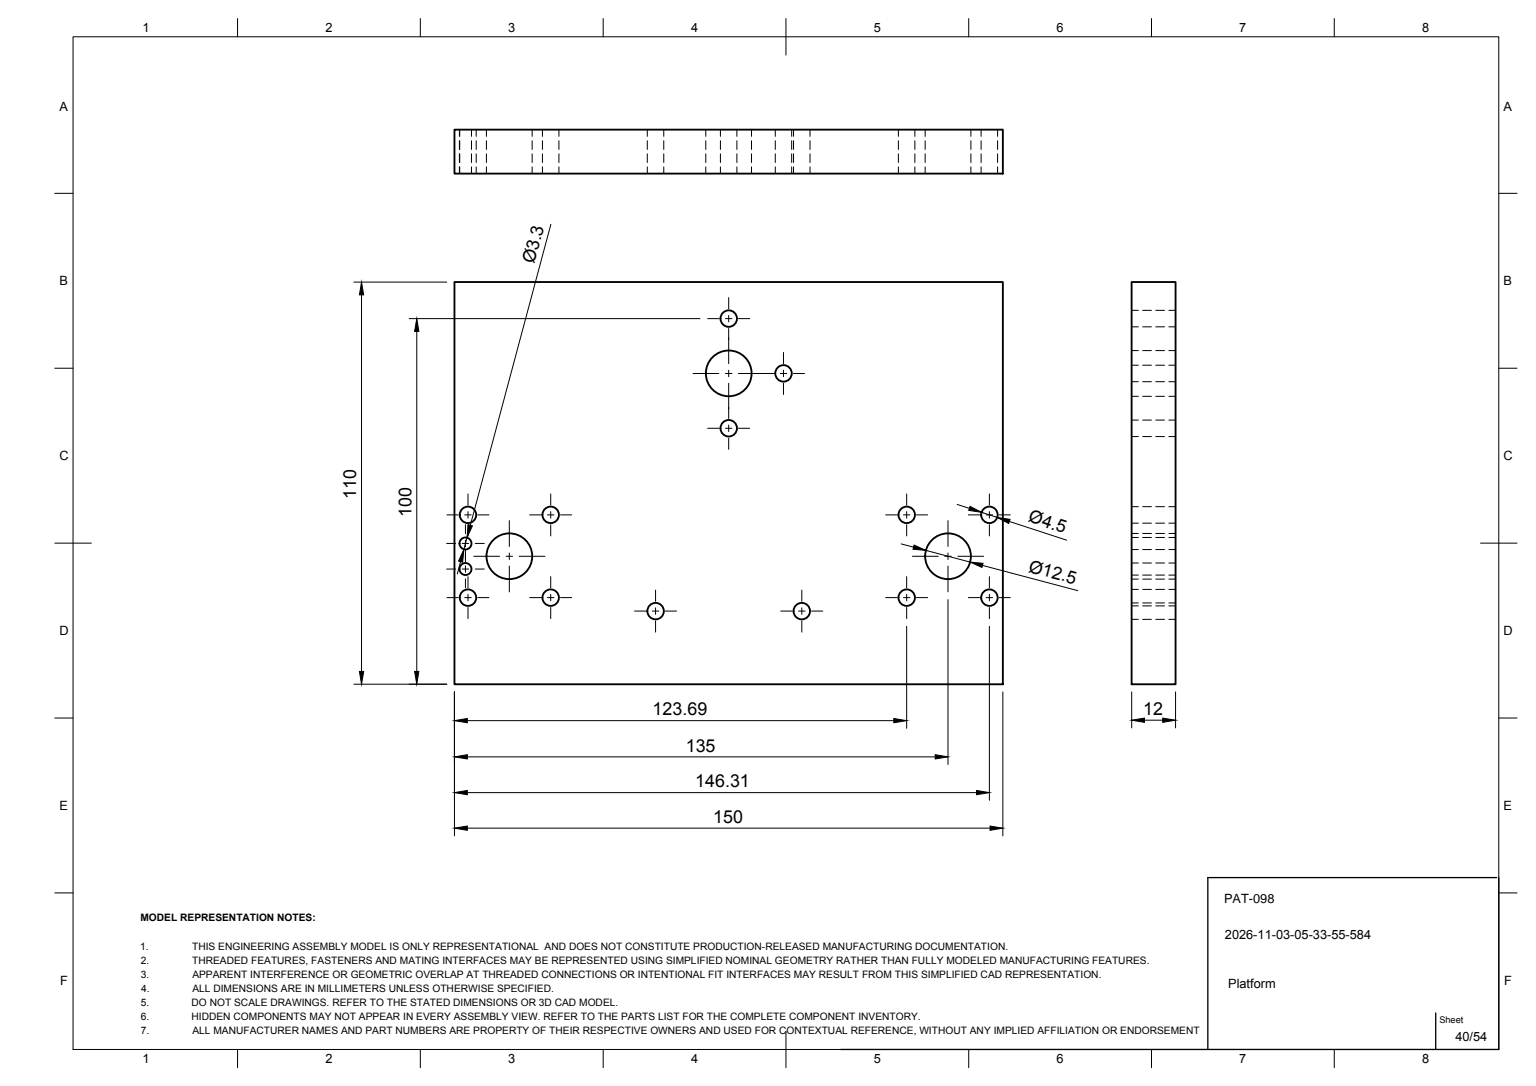
ISO-10303-21;
HEADER;
/* Generated by software containing ST-Developer
 * from STEP Tools, Inc. (www.steptools.com) 
 */

FILE_DESCRIPTION(
/* description */ ('Spring compression tester'),
/* implementation_level */ '2;1');

FILE_NAME(
/* name */ 'Platform.step',
/* time_stamp */ '2026-10-28T03:24:11-07:00',
/* author */ (''),
/* organization */ (''),
/* preprocessor_version */ 'ST-DEVELOPER v20.2',
/* originating_system */ 'Autodesk Translation Framework v15.17.0.0',
/* authorisation */ '');

FILE_SCHEMA (('AUTOMOTIVE_DESIGN { 1 0 10303 214 3 1 1 }'));
ENDSEC;

DATA;
#10=MECHANICAL_DESIGN_GEOMETRIC_PRESENTATION_REPRESENTATION('',(#1158),#43521);
#1023=SHAPE_REPRESENTATION_RELATIONSHIP('SRR','None',#43838,#1083);
#1083=ADVANCED_BREP_SHAPE_REPRESENTATION('',(#1229),#43498);
#1158=STYLED_ITEM('',(#44188),#1229);
#1229=MANIFOLD_SOLID_BREP('Body1',#18599);
#1477=FACE_BOUND('',#4122,.T.);
#1478=FACE_BOUND('',#4123,.T.);
#1479=FACE_BOUND('',#4124,.T.);
#1480=FACE_BOUND('',#4125,.T.);
#1481=FACE_BOUND('',#4126,.T.);
#1482=FACE_BOUND('',#4127,.T.);
#1483=FACE_BOUND('',#4128,.T.);
#1484=FACE_BOUND('',#4129,.T.);
#1485=FACE_BOUND('',#4130,.T.);
#1486=FACE_BOUND('',#4131,.T.);
#1487=FACE_BOUND('',#4132,.T.);
#1488=FACE_BOUND('',#4133,.T.);
#1489=FACE_BOUND('',#4134,.T.);
#1490=FACE_BOUND('',#4135,.T.);
#1491=FACE_BOUND('',#4136,.T.);
#1492=FACE_BOUND('',#4137,.T.);
#1493=FACE_BOUND('',#4138,.T.);
#1494=FACE_BOUND('',#4139,.T.);
#1495=FACE_BOUND('',#4141,.T.);
#1496=FACE_BOUND('',#4142,.T.);
#1497=FACE_BOUND('',#4143,.T.);
#1498=FACE_BOUND('',#4144,.T.);
#1499=FACE_BOUND('',#4145,.T.);
#1500=FACE_BOUND('',#4146,.T.);
#1501=FACE_BOUND('',#4147,.T.);
#1502=FACE_BOUND('',#4148,.T.);
#1503=FACE_BOUND('',#4149,.T.);
#1504=FACE_BOUND('',#4150,.T.);
#1505=FACE_BOUND('',#4151,.T.);
#1506=FACE_BOUND('',#4152,.T.);
#1507=FACE_BOUND('',#4153,.T.);
#1508=FACE_BOUND('',#4154,.T.);
#1509=FACE_BOUND('',#4155,.T.);
#1510=FACE_BOUND('',#4156,.T.);
#1511=FACE_BOUND('',#4157,.T.);
#1512=FACE_BOUND('',#4158,.T.);
#2024=PLANE('',#20482);
#2025=PLANE('',#20483);
#2026=PLANE('',#20484);
#2027=PLANE('',#20485);
#2028=PLANE('',#20486);
#2029=PLANE('',#20487);
#2822=FACE_OUTER_BOUND('',#4099,.T.);
#2823=FACE_OUTER_BOUND('',#4100,.T.);
#2824=FACE_OUTER_BOUND('',#4101,.T.);
#2825=FACE_OUTER_BOUND('',#4102,.T.);
#2826=FACE_OUTER_BOUND('',#4103,.T.);
#2827=FACE_OUTER_BOUND('',#4104,.T.);
#2828=FACE_OUTER_BOUND('',#4105,.T.);
#2829=FACE_OUTER_BOUND('',#4106,.T.);
#2830=FACE_OUTER_BOUND('',#4107,.T.);
#2831=FACE_OUTER_BOUND('',#4108,.T.);
#2832=FACE_OUTER_BOUND('',#4109,.T.);
#2833=FACE_OUTER_BOUND('',#4110,.T.);
#2834=FACE_OUTER_BOUND('',#4111,.T.);
#2835=FACE_OUTER_BOUND('',#4112,.T.);
#2836=FACE_OUTER_BOUND('',#4113,.T.);
#2837=FACE_OUTER_BOUND('',#4114,.T.);
#2838=FACE_OUTER_BOUND('',#4115,.T.);
#2839=FACE_OUTER_BOUND('',#4116,.T.);
#2840=FACE_OUTER_BOUND('',#4117,.T.);
#2841=FACE_OUTER_BOUND('',#4118,.T.);
#2842=FACE_OUTER_BOUND('',#4119,.T.);
#2843=FACE_OUTER_BOUND('',#4120,.T.);
#2844=FACE_OUTER_BOUND('',#4121,.T.);
#2845=FACE_OUTER_BOUND('',#4140,.T.);
#4099=EDGE_LOOP('',(#15129,#15130,#15131,#15132));
#4100=EDGE_LOOP('',(#15133,#15134,#15135,#15136));
#4101=EDGE_LOOP('',(#15137,#15138,#15139,#15140));
#4102=EDGE_LOOP('',(#15141,#15142,#15143,#15144));
#4103=EDGE_LOOP('',(#15145,#15146,#15147,#15148));
#4104=EDGE_LOOP('',(#15149,#15150,#15151,#15152));
#4105=EDGE_LOOP('',(#15153,#15154,#15155,#15156));
#4106=EDGE_LOOP('',(#15157,#15158,#15159,#15160));
#4107=EDGE_LOOP('',(#15161,#15162,#15163,#15164));
#4108=EDGE_LOOP('',(#15165,#15166,#15167,#15168));
#4109=EDGE_LOOP('',(#15169,#15170,#15171,#15172));
#4110=EDGE_LOOP('',(#15173,#15174,#15175,#15176));
#4111=EDGE_LOOP('',(#15177,#15178,#15179,#15180));
#4112=EDGE_LOOP('',(#15181,#15182,#15183,#15184));
#4113=EDGE_LOOP('',(#15185,#15186,#15187,#15188));
#4114=EDGE_LOOP('',(#15189,#15190,#15191,#15192));
#4115=EDGE_LOOP('',(#15193,#15194,#15195,#15196));
#4116=EDGE_LOOP('',(#15197,#15198,#15199,#15200));
#4117=EDGE_LOOP('',(#15201,#15202,#15203,#15204));
#4118=EDGE_LOOP('',(#15205,#15206,#15207,#15208));
#4119=EDGE_LOOP('',(#15209,#15210,#15211,#15212));
#4120=EDGE_LOOP('',(#15213,#15214,#15215,#15216));
#4121=EDGE_LOOP('',(#15217,#15218,#15219,#15220));
#4122=EDGE_LOOP('',(#15221));
#4123=EDGE_LOOP('',(#15222));
#4124=EDGE_LOOP('',(#15223));
#4125=EDGE_LOOP('',(#15224));
#4126=EDGE_LOOP('',(#15225));
#4127=EDGE_LOOP('',(#15226));
#4128=EDGE_LOOP('',(#15227));
#4129=EDGE_LOOP('',(#15228));
#4130=EDGE_LOOP('',(#15229));
#4131=EDGE_LOOP('',(#15230));
#4132=EDGE_LOOP('',(#15231));
#4133=EDGE_LOOP('',(#15232));
#4134=EDGE_LOOP('',(#15233));
#4135=EDGE_LOOP('',(#15234));
#4136=EDGE_LOOP('',(#15235));
#4137=EDGE_LOOP('',(#15236));
#4138=EDGE_LOOP('',(#15237));
#4139=EDGE_LOOP('',(#15238));
#4140=EDGE_LOOP('',(#15239,#15240,#15241,#15242));
#4141=EDGE_LOOP('',(#15243));
#4142=EDGE_LOOP('',(#15244));
#4143=EDGE_LOOP('',(#15245));
#4144=EDGE_LOOP('',(#15246));
#4145=EDGE_LOOP('',(#15247));
#4146=EDGE_LOOP('',(#15248));
#4147=EDGE_LOOP('',(#15249));
#4148=EDGE_LOOP('',(#15250));
#4149=EDGE_LOOP('',(#15251));
#4150=EDGE_LOOP('',(#15252));
#4151=EDGE_LOOP('',(#15253));
#4152=EDGE_LOOP('',(#15254));
#4153=EDGE_LOOP('',(#15255));
#4154=EDGE_LOOP('',(#15256));
#4155=EDGE_LOOP('',(#15257));
#4156=EDGE_LOOP('',(#15258));
#4157=EDGE_LOOP('',(#15259));
#4158=EDGE_LOOP('',(#15260));
#5593=LINE('',#30233,#7025);
#5594=LINE('',#30239,#7026);
#5595=LINE('',#30245,#7027);
#5596=LINE('',#30251,#7028);
#5597=LINE('',#30257,#7029);
#5598=LINE('',#30263,#7030);
#5599=LINE('',#30269,#7031);
#5600=LINE('',#30275,#7032);
#5601=LINE('',#30281,#7033);
#5602=LINE('',#30287,#7034);
#5603=LINE('',#30293,#7035);
#5604=LINE('',#30299,#7036);
#5605=LINE('',#30305,#7037);
#5606=LINE('',#30311,#7038);
#5607=LINE('',#30317,#7039);
#5608=LINE('',#30323,#7040);
#5609=LINE('',#30329,#7041);
#5610=LINE('',#30335,#7042);
#5611=LINE('',#30340,#7043);
#5612=LINE('',#30342,#7044);
#5613=LINE('',#30344,#7045);
#5614=LINE('',#30345,#7046);
#5615=LINE('',#30348,#7047);
#5616=LINE('',#30350,#7048);
#5617=LINE('',#30351,#7049);
#5618=LINE('',#30354,#7050);
#5619=LINE('',#30356,#7051);
#5620=LINE('',#30357,#7052);
#5621=LINE('',#30359,#7053);
#5622=LINE('',#30360,#7054);
#7025=VECTOR('',#24475,0.165);
#7026=VECTOR('',#24482,0.165);
#7027=VECTOR('',#24489,0.225);
#7028=VECTOR('',#24496,0.225);
#7029=VECTOR('',#24503,0.225);
#7030=VECTOR('',#24510,0.225);
#7031=VECTOR('',#24517,0.225);
#7032=VECTOR('',#24524,0.225);
#7033=VECTOR('',#24531,0.225);
#7034=VECTOR('',#24538,0.225);
#7035=VECTOR('',#24545,0.225);
#7036=VECTOR('',#24552,0.225);
#7037=VECTOR('',#24559,0.225);
#7038=VECTOR('',#24566,0.225);
#7039=VECTOR('',#24573,0.225);
#7040=VECTOR('',#24580,0.625);
#7041=VECTOR('',#24587,0.625);
#7042=VECTOR('',#24594,0.625);
#7043=VECTOR('',#24599,1.);
#7044=VECTOR('',#24600,1.);
#7045=VECTOR('',#24601,1.);
#7046=VECTOR('',#24602,1.);
#7047=VECTOR('',#24605,1.);
#7048=VECTOR('',#24606,1.);
#7049=VECTOR('',#24607,1.);
#7050=VECTOR('',#24610,1.);
#7051=VECTOR('',#24611,1.);
#7052=VECTOR('',#24612,1.);
#7053=VECTOR('',#24615,1.);
#7054=VECTOR('',#24616,1.);
#7905=CIRCLE('',#20429,0.165);
#7906=CIRCLE('',#20430,0.165);
#7907=CIRCLE('',#20432,0.165);
#7908=CIRCLE('',#20433,0.165);
#7909=CIRCLE('',#20435,0.225);
#7910=CIRCLE('',#20436,0.225);
#7911=CIRCLE('',#20438,0.225);
#7912=CIRCLE('',#20439,0.225);
#7913=CIRCLE('',#20441,0.225);
#7914=CIRCLE('',#20442,0.225);
#7915=CIRCLE('',#20444,0.225);
#7916=CIRCLE('',#20445,0.225);
#7917=CIRCLE('',#20447,0.225);
#7918=CIRCLE('',#20448,0.225);
#7919=CIRCLE('',#20450,0.225);
#7920=CIRCLE('',#20451,0.225);
#7921=CIRCLE('',#20453,0.225);
#7922=CIRCLE('',#20454,0.225);
#7923=CIRCLE('',#20456,0.225);
#7924=CIRCLE('',#20457,0.225);
#7925=CIRCLE('',#20459,0.225);
#7926=CIRCLE('',#20460,0.225);
#7927=CIRCLE('',#20462,0.225);
#7928=CIRCLE('',#20463,0.225);
#7929=CIRCLE('',#20465,0.225);
#7930=CIRCLE('',#20466,0.225);
#7931=CIRCLE('',#20468,0.225);
#7932=CIRCLE('',#20469,0.225);
#7933=CIRCLE('',#20471,0.225);
#7934=CIRCLE('',#20472,0.225);
#7935=CIRCLE('',#20474,0.625);
#7936=CIRCLE('',#20475,0.625);
#7937=CIRCLE('',#20477,0.625);
#7938=CIRCLE('',#20478,0.625);
#7939=CIRCLE('',#20480,0.625);
#7940=CIRCLE('',#20481,0.625);
#9118=VERTEX_POINT('',#30230);
#9119=VERTEX_POINT('',#30232);
#9120=VERTEX_POINT('',#30236);
#9121=VERTEX_POINT('',#30238);
#9122=VERTEX_POINT('',#30242);
#9123=VERTEX_POINT('',#30244);
#9124=VERTEX_POINT('',#30248);
#9125=VERTEX_POINT('',#30250);
#9126=VERTEX_POINT('',#30254);
#9127=VERTEX_POINT('',#30256);
#9128=VERTEX_POINT('',#30260);
#9129=VERTEX_POINT('',#30262);
#9130=VERTEX_POINT('',#30266);
#9131=VERTEX_POINT('',#30268);
#9132=VERTEX_POINT('',#30272);
#9133=VERTEX_POINT('',#30274);
#9134=VERTEX_POINT('',#30278);
#9135=VERTEX_POINT('',#30280);
#9136=VERTEX_POINT('',#30284);
#9137=VERTEX_POINT('',#30286);
#9138=VERTEX_POINT('',#30290);
#9139=VERTEX_POINT('',#30292);
#9140=VERTEX_POINT('',#30296);
#9141=VERTEX_POINT('',#30298);
#9142=VERTEX_POINT('',#30302);
#9143=VERTEX_POINT('',#30304);
#9144=VERTEX_POINT('',#30308);
#9145=VERTEX_POINT('',#30310);
#9146=VERTEX_POINT('',#30314);
#9147=VERTEX_POINT('',#30316);
#9148=VERTEX_POINT('',#30320);
#9149=VERTEX_POINT('',#30322);
#9150=VERTEX_POINT('',#30326);
#9151=VERTEX_POINT('',#30328);
#9152=VERTEX_POINT('',#30332);
#9153=VERTEX_POINT('',#30334);
#9154=VERTEX_POINT('',#30338);
#9155=VERTEX_POINT('',#30339);
#9156=VERTEX_POINT('',#30341);
#9157=VERTEX_POINT('',#30343);
#9158=VERTEX_POINT('',#30347);
#9159=VERTEX_POINT('',#30349);
#9160=VERTEX_POINT('',#30353);
#9161=VERTEX_POINT('',#30355);
#11229=EDGE_CURVE('',#9118,#9118,#7905,.T.);
#11230=EDGE_CURVE('',#9118,#9119,#5593,.T.);
#11231=EDGE_CURVE('',#9119,#9119,#7906,.T.);
#11232=EDGE_CURVE('',#9120,#9120,#7907,.T.);
#11233=EDGE_CURVE('',#9120,#9121,#5594,.T.);
#11234=EDGE_CURVE('',#9121,#9121,#7908,.T.);
#11235=EDGE_CURVE('',#9122,#9122,#7909,.T.);
#11236=EDGE_CURVE('',#9122,#9123,#5595,.T.);
#11237=EDGE_CURVE('',#9123,#9123,#7910,.T.);
#11238=EDGE_CURVE('',#9124,#9124,#7911,.T.);
#11239=EDGE_CURVE('',#9124,#9125,#5596,.T.);
#11240=EDGE_CURVE('',#9125,#9125,#7912,.T.);
#11241=EDGE_CURVE('',#9126,#9126,#7913,.T.);
#11242=EDGE_CURVE('',#9126,#9127,#5597,.T.);
#11243=EDGE_CURVE('',#9127,#9127,#7914,.T.);
#11244=EDGE_CURVE('',#9128,#9128,#7915,.T.);
#11245=EDGE_CURVE('',#9128,#9129,#5598,.T.);
#11246=EDGE_CURVE('',#9129,#9129,#7916,.T.);
#11247=EDGE_CURVE('',#9130,#9130,#7917,.T.);
#11248=EDGE_CURVE('',#9130,#9131,#5599,.T.);
#11249=EDGE_CURVE('',#9131,#9131,#7918,.T.);
#11250=EDGE_CURVE('',#9132,#9132,#7919,.T.);
#11251=EDGE_CURVE('',#9132,#9133,#5600,.T.);
#11252=EDGE_CURVE('',#9133,#9133,#7920,.T.);
#11253=EDGE_CURVE('',#9134,#9134,#7921,.T.);
#11254=EDGE_CURVE('',#9134,#9135,#5601,.T.);
#11255=EDGE_CURVE('',#9135,#9135,#7922,.T.);
#11256=EDGE_CURVE('',#9136,#9136,#7923,.T.);
#11257=EDGE_CURVE('',#9136,#9137,#5602,.T.);
#11258=EDGE_CURVE('',#9137,#9137,#7924,.T.);
#11259=EDGE_CURVE('',#9138,#9138,#7925,.T.);
#11260=EDGE_CURVE('',#9138,#9139,#5603,.T.);
#11261=EDGE_CURVE('',#9139,#9139,#7926,.T.);
#11262=EDGE_CURVE('',#9140,#9140,#7927,.T.);
#11263=EDGE_CURVE('',#9140,#9141,#5604,.T.);
#11264=EDGE_CURVE('',#9141,#9141,#7928,.T.);
#11265=EDGE_CURVE('',#9142,#9142,#7929,.T.);
#11266=EDGE_CURVE('',#9142,#9143,#5605,.T.);
#11267=EDGE_CURVE('',#9143,#9143,#7930,.T.);
#11268=EDGE_CURVE('',#9144,#9144,#7931,.T.);
#11269=EDGE_CURVE('',#9144,#9145,#5606,.T.);
#11270=EDGE_CURVE('',#9145,#9145,#7932,.T.);
#11271=EDGE_CURVE('',#9146,#9146,#7933,.T.);
#11272=EDGE_CURVE('',#9146,#9147,#5607,.T.);
#11273=EDGE_CURVE('',#9147,#9147,#7934,.T.);
#11274=EDGE_CURVE('',#9148,#9148,#7935,.T.);
#11275=EDGE_CURVE('',#9148,#9149,#5608,.T.);
#11276=EDGE_CURVE('',#9149,#9149,#7936,.T.);
#11277=EDGE_CURVE('',#9150,#9150,#7937,.T.);
#11278=EDGE_CURVE('',#9150,#9151,#5609,.T.);
#11279=EDGE_CURVE('',#9151,#9151,#7938,.T.);
#11280=EDGE_CURVE('',#9152,#9152,#7939,.T.);
#11281=EDGE_CURVE('',#9152,#9153,#5610,.T.);
#11282=EDGE_CURVE('',#9153,#9153,#7940,.T.);
#11283=EDGE_CURVE('',#9154,#9155,#5611,.T.);
#11284=EDGE_CURVE('',#9155,#9156,#5612,.T.);
#11285=EDGE_CURVE('',#9157,#9156,#5613,.T.);
#11286=EDGE_CURVE('',#9154,#9157,#5614,.T.);
#11287=EDGE_CURVE('',#9158,#9154,#5615,.T.);
#11288=EDGE_CURVE('',#9159,#9157,#5616,.T.);
#11289=EDGE_CURVE('',#9158,#9159,#5617,.T.);
#11290=EDGE_CURVE('',#9160,#9158,#5618,.T.);
#11291=EDGE_CURVE('',#9161,#9159,#5619,.T.);
#11292=EDGE_CURVE('',#9160,#9161,#5620,.T.);
#11293=EDGE_CURVE('',#9155,#9160,#5621,.T.);
#11294=EDGE_CURVE('',#9156,#9161,#5622,.T.);
#15129=ORIENTED_EDGE('',*,*,#11229,.F.);
#15130=ORIENTED_EDGE('',*,*,#11230,.T.);
#15131=ORIENTED_EDGE('',*,*,#11231,.F.);
#15132=ORIENTED_EDGE('',*,*,#11230,.F.);
#15133=ORIENTED_EDGE('',*,*,#11232,.F.);
#15134=ORIENTED_EDGE('',*,*,#11233,.T.);
#15135=ORIENTED_EDGE('',*,*,#11234,.F.);
#15136=ORIENTED_EDGE('',*,*,#11233,.F.);
#15137=ORIENTED_EDGE('',*,*,#11235,.F.);
#15138=ORIENTED_EDGE('',*,*,#11236,.T.);
#15139=ORIENTED_EDGE('',*,*,#11237,.F.);
#15140=ORIENTED_EDGE('',*,*,#11236,.F.);
#15141=ORIENTED_EDGE('',*,*,#11238,.F.);
#15142=ORIENTED_EDGE('',*,*,#11239,.T.);
#15143=ORIENTED_EDGE('',*,*,#11240,.F.);
#15144=ORIENTED_EDGE('',*,*,#11239,.F.);
#15145=ORIENTED_EDGE('',*,*,#11241,.F.);
#15146=ORIENTED_EDGE('',*,*,#11242,.T.);
#15147=ORIENTED_EDGE('',*,*,#11243,.F.);
#15148=ORIENTED_EDGE('',*,*,#11242,.F.);
#15149=ORIENTED_EDGE('',*,*,#11244,.F.);
#15150=ORIENTED_EDGE('',*,*,#11245,.T.);
#15151=ORIENTED_EDGE('',*,*,#11246,.F.);
#15152=ORIENTED_EDGE('',*,*,#11245,.F.);
#15153=ORIENTED_EDGE('',*,*,#11247,.F.);
#15154=ORIENTED_EDGE('',*,*,#11248,.T.);
#15155=ORIENTED_EDGE('',*,*,#11249,.F.);
#15156=ORIENTED_EDGE('',*,*,#11248,.F.);
#15157=ORIENTED_EDGE('',*,*,#11250,.F.);
#15158=ORIENTED_EDGE('',*,*,#11251,.T.);
#15159=ORIENTED_EDGE('',*,*,#11252,.F.);
#15160=ORIENTED_EDGE('',*,*,#11251,.F.);
#15161=ORIENTED_EDGE('',*,*,#11253,.F.);
#15162=ORIENTED_EDGE('',*,*,#11254,.T.);
#15163=ORIENTED_EDGE('',*,*,#11255,.F.);
#15164=ORIENTED_EDGE('',*,*,#11254,.F.);
#15165=ORIENTED_EDGE('',*,*,#11256,.F.);
#15166=ORIENTED_EDGE('',*,*,#11257,.T.);
#15167=ORIENTED_EDGE('',*,*,#11258,.F.);
#15168=ORIENTED_EDGE('',*,*,#11257,.F.);
#15169=ORIENTED_EDGE('',*,*,#11259,.F.);
#15170=ORIENTED_EDGE('',*,*,#11260,.T.);
#15171=ORIENTED_EDGE('',*,*,#11261,.F.);
#15172=ORIENTED_EDGE('',*,*,#11260,.F.);
#15173=ORIENTED_EDGE('',*,*,#11262,.F.);
#15174=ORIENTED_EDGE('',*,*,#11263,.T.);
#15175=ORIENTED_EDGE('',*,*,#11264,.F.);
#15176=ORIENTED_EDGE('',*,*,#11263,.F.);
#15177=ORIENTED_EDGE('',*,*,#11265,.F.);
#15178=ORIENTED_EDGE('',*,*,#11266,.T.);
#15179=ORIENTED_EDGE('',*,*,#11267,.F.);
#15180=ORIENTED_EDGE('',*,*,#11266,.F.);
#15181=ORIENTED_EDGE('',*,*,#11268,.F.);
#15182=ORIENTED_EDGE('',*,*,#11269,.T.);
#15183=ORIENTED_EDGE('',*,*,#11270,.F.);
#15184=ORIENTED_EDGE('',*,*,#11269,.F.);
#15185=ORIENTED_EDGE('',*,*,#11271,.F.);
#15186=ORIENTED_EDGE('',*,*,#11272,.T.);
#15187=ORIENTED_EDGE('',*,*,#11273,.F.);
#15188=ORIENTED_EDGE('',*,*,#11272,.F.);
#15189=ORIENTED_EDGE('',*,*,#11274,.F.);
#15190=ORIENTED_EDGE('',*,*,#11275,.T.);
#15191=ORIENTED_EDGE('',*,*,#11276,.F.);
#15192=ORIENTED_EDGE('',*,*,#11275,.F.);
#15193=ORIENTED_EDGE('',*,*,#11277,.F.);
#15194=ORIENTED_EDGE('',*,*,#11278,.T.);
#15195=ORIENTED_EDGE('',*,*,#11279,.F.);
#15196=ORIENTED_EDGE('',*,*,#11278,.F.);
#15197=ORIENTED_EDGE('',*,*,#11280,.F.);
#15198=ORIENTED_EDGE('',*,*,#11281,.T.);
#15199=ORIENTED_EDGE('',*,*,#11282,.F.);
#15200=ORIENTED_EDGE('',*,*,#11281,.F.);
#15201=ORIENTED_EDGE('',*,*,#11283,.T.);
#15202=ORIENTED_EDGE('',*,*,#11284,.T.);
#15203=ORIENTED_EDGE('',*,*,#11285,.F.);
#15204=ORIENTED_EDGE('',*,*,#11286,.F.);
#15205=ORIENTED_EDGE('',*,*,#11287,.T.);
#15206=ORIENTED_EDGE('',*,*,#11286,.T.);
#15207=ORIENTED_EDGE('',*,*,#11288,.F.);
#15208=ORIENTED_EDGE('',*,*,#11289,.F.);
#15209=ORIENTED_EDGE('',*,*,#11290,.T.);
#15210=ORIENTED_EDGE('',*,*,#11289,.T.);
#15211=ORIENTED_EDGE('',*,*,#11291,.F.);
#15212=ORIENTED_EDGE('',*,*,#11292,.F.);
#15213=ORIENTED_EDGE('',*,*,#11293,.T.);
#15214=ORIENTED_EDGE('',*,*,#11292,.T.);
#15215=ORIENTED_EDGE('',*,*,#11294,.F.);
#15216=ORIENTED_EDGE('',*,*,#11284,.F.);
#15217=ORIENTED_EDGE('',*,*,#11294,.T.);
#15218=ORIENTED_EDGE('',*,*,#11291,.T.);
#15219=ORIENTED_EDGE('',*,*,#11288,.T.);
#15220=ORIENTED_EDGE('',*,*,#11285,.T.);
#15221=ORIENTED_EDGE('',*,*,#11237,.T.);
#15222=ORIENTED_EDGE('',*,*,#11240,.T.);
#15223=ORIENTED_EDGE('',*,*,#11252,.T.);
#15224=ORIENTED_EDGE('',*,*,#11255,.T.);
#15225=ORIENTED_EDGE('',*,*,#11258,.T.);
#15226=ORIENTED_EDGE('',*,*,#11261,.T.);
#15227=ORIENTED_EDGE('',*,*,#11282,.T.);
#15228=ORIENTED_EDGE('',*,*,#11279,.T.);
#15229=ORIENTED_EDGE('',*,*,#11276,.T.);
#15230=ORIENTED_EDGE('',*,*,#11273,.T.);
#15231=ORIENTED_EDGE('',*,*,#11270,.T.);
#15232=ORIENTED_EDGE('',*,*,#11267,.T.);
#15233=ORIENTED_EDGE('',*,*,#11264,.T.);
#15234=ORIENTED_EDGE('',*,*,#11249,.T.);
#15235=ORIENTED_EDGE('',*,*,#11246,.T.);
#15236=ORIENTED_EDGE('',*,*,#11243,.T.);
#15237=ORIENTED_EDGE('',*,*,#11234,.T.);
#15238=ORIENTED_EDGE('',*,*,#11231,.T.);
#15239=ORIENTED_EDGE('',*,*,#11293,.F.);
#15240=ORIENTED_EDGE('',*,*,#11283,.F.);
#15241=ORIENTED_EDGE('',*,*,#11287,.F.);
#15242=ORIENTED_EDGE('',*,*,#11290,.F.);
#15243=ORIENTED_EDGE('',*,*,#11235,.T.);
#15244=ORIENTED_EDGE('',*,*,#11238,.T.);
#15245=ORIENTED_EDGE('',*,*,#11250,.T.);
#15246=ORIENTED_EDGE('',*,*,#11253,.T.);
#15247=ORIENTED_EDGE('',*,*,#11256,.T.);
#15248=ORIENTED_EDGE('',*,*,#11259,.T.);
#15249=ORIENTED_EDGE('',*,*,#11280,.T.);
#15250=ORIENTED_EDGE('',*,*,#11277,.T.);
#15251=ORIENTED_EDGE('',*,*,#11274,.T.);
#15252=ORIENTED_EDGE('',*,*,#11271,.T.);
#15253=ORIENTED_EDGE('',*,*,#11268,.T.);
#15254=ORIENTED_EDGE('',*,*,#11265,.T.);
#15255=ORIENTED_EDGE('',*,*,#11262,.T.);
#15256=ORIENTED_EDGE('',*,*,#11247,.T.);
#15257=ORIENTED_EDGE('',*,*,#11244,.T.);
#15258=ORIENTED_EDGE('',*,*,#11241,.T.);
#15259=ORIENTED_EDGE('',*,*,#11232,.T.);
#15260=ORIENTED_EDGE('',*,*,#11229,.T.);
#17262=CYLINDRICAL_SURFACE('',#20428,0.165);
#17263=CYLINDRICAL_SURFACE('',#20431,0.165);
#17264=CYLINDRICAL_SURFACE('',#20434,0.225);
#17265=CYLINDRICAL_SURFACE('',#20437,0.225);
#17266=CYLINDRICAL_SURFACE('',#20440,0.225);
#17267=CYLINDRICAL_SURFACE('',#20443,0.225);
#17268=CYLINDRICAL_SURFACE('',#20446,0.225);
#17269=CYLINDRICAL_SURFACE('',#20449,0.225);
#17270=CYLINDRICAL_SURFACE('',#20452,0.225);
#17271=CYLINDRICAL_SURFACE('',#20455,0.225);
#17272=CYLINDRICAL_SURFACE('',#20458,0.225);
#17273=CYLINDRICAL_SURFACE('',#20461,0.225);
#17274=CYLINDRICAL_SURFACE('',#20464,0.225);
#17275=CYLINDRICAL_SURFACE('',#20467,0.225);
#17276=CYLINDRICAL_SURFACE('',#20470,0.225);
#17277=CYLINDRICAL_SURFACE('',#20473,0.625);
#17278=CYLINDRICAL_SURFACE('',#20476,0.625);
#17279=CYLINDRICAL_SURFACE('',#20479,0.625);
#18146=ADVANCED_FACE('',(#2822),#17262,.F.);
#18147=ADVANCED_FACE('',(#2823),#17263,.F.);
#18148=ADVANCED_FACE('',(#2824),#17264,.F.);
#18149=ADVANCED_FACE('',(#2825),#17265,.F.);
#18150=ADVANCED_FACE('',(#2826),#17266,.F.);
#18151=ADVANCED_FACE('',(#2827),#17267,.F.);
#18152=ADVANCED_FACE('',(#2828),#17268,.F.);
#18153=ADVANCED_FACE('',(#2829),#17269,.F.);
#18154=ADVANCED_FACE('',(#2830),#17270,.F.);
#18155=ADVANCED_FACE('',(#2831),#17271,.F.);
#18156=ADVANCED_FACE('',(#2832),#17272,.F.);
#18157=ADVANCED_FACE('',(#2833),#17273,.F.);
#18158=ADVANCED_FACE('',(#2834),#17274,.F.);
#18159=ADVANCED_FACE('',(#2835),#17275,.F.);
#18160=ADVANCED_FACE('',(#2836),#17276,.F.);
#18161=ADVANCED_FACE('',(#2837),#17277,.F.);
#18162=ADVANCED_FACE('',(#2838),#17278,.F.);
#18163=ADVANCED_FACE('',(#2839),#17279,.F.);
#18164=ADVANCED_FACE('',(#2840),#2024,.T.);
#18165=ADVANCED_FACE('',(#2841),#2025,.T.);
#18166=ADVANCED_FACE('',(#2842),#2026,.T.);
#18167=ADVANCED_FACE('',(#2843),#2027,.T.);
#18168=ADVANCED_FACE('',(#2844,#1477,#1478,#1479,#1480,#1481,#1482,#1483,
#1484,#1485,#1486,#1487,#1488,#1489,#1490,#1491,#1492,#1493,#1494),#2028,
 .T.);
#18169=ADVANCED_FACE('',(#2845,#1495,#1496,#1497,#1498,#1499,#1500,#1501,
#1502,#1503,#1504,#1505,#1506,#1507,#1508,#1509,#1510,#1511,#1512),#2029,
 .F.);
#18599=CLOSED_SHELL('',(#18146,#18147,#18148,#18149,#18150,#18151,#18152,
#18153,#18154,#18155,#18156,#18157,#18158,#18159,#18160,#18161,#18162,#18163,
#18164,#18165,#18166,#18167,#18168,#18169));
#20427=AXIS2_PLACEMENT_3D('',#30228,#24469,#24470);
#20428=AXIS2_PLACEMENT_3D('',#30229,#24471,#24472);
#20429=AXIS2_PLACEMENT_3D('',#30231,#24473,#24474);
#20430=AXIS2_PLACEMENT_3D('',#30234,#24476,#24477);
#20431=AXIS2_PLACEMENT_3D('',#30235,#24478,#24479);
#20432=AXIS2_PLACEMENT_3D('',#30237,#24480,#24481);
#20433=AXIS2_PLACEMENT_3D('',#30240,#24483,#24484);
#20434=AXIS2_PLACEMENT_3D('',#30241,#24485,#24486);
#20435=AXIS2_PLACEMENT_3D('',#30243,#24487,#24488);
#20436=AXIS2_PLACEMENT_3D('',#30246,#24490,#24491);
#20437=AXIS2_PLACEMENT_3D('',#30247,#24492,#24493);
#20438=AXIS2_PLACEMENT_3D('',#30249,#24494,#24495);
#20439=AXIS2_PLACEMENT_3D('',#30252,#24497,#24498);
#20440=AXIS2_PLACEMENT_3D('',#30253,#24499,#24500);
#20441=AXIS2_PLACEMENT_3D('',#30255,#24501,#24502);
#20442=AXIS2_PLACEMENT_3D('',#30258,#24504,#24505);
#20443=AXIS2_PLACEMENT_3D('',#30259,#24506,#24507);
#20444=AXIS2_PLACEMENT_3D('',#30261,#24508,#24509);
#20445=AXIS2_PLACEMENT_3D('',#30264,#24511,#24512);
#20446=AXIS2_PLACEMENT_3D('',#30265,#24513,#24514);
#20447=AXIS2_PLACEMENT_3D('',#30267,#24515,#24516);
#20448=AXIS2_PLACEMENT_3D('',#30270,#24518,#24519);
#20449=AXIS2_PLACEMENT_3D('',#30271,#24520,#24521);
#20450=AXIS2_PLACEMENT_3D('',#30273,#24522,#24523);
#20451=AXIS2_PLACEMENT_3D('',#30276,#24525,#24526);
#20452=AXIS2_PLACEMENT_3D('',#30277,#24527,#24528);
#20453=AXIS2_PLACEMENT_3D('',#30279,#24529,#24530);
#20454=AXIS2_PLACEMENT_3D('',#30282,#24532,#24533);
#20455=AXIS2_PLACEMENT_3D('',#30283,#24534,#24535);
#20456=AXIS2_PLACEMENT_3D('',#30285,#24536,#24537);
#20457=AXIS2_PLACEMENT_3D('',#30288,#24539,#24540);
#20458=AXIS2_PLACEMENT_3D('',#30289,#24541,#24542);
#20459=AXIS2_PLACEMENT_3D('',#30291,#24543,#24544);
#20460=AXIS2_PLACEMENT_3D('',#30294,#24546,#24547);
#20461=AXIS2_PLACEMENT_3D('',#30295,#24548,#24549);
#20462=AXIS2_PLACEMENT_3D('',#30297,#24550,#24551);
#20463=AXIS2_PLACEMENT_3D('',#30300,#24553,#24554);
#20464=AXIS2_PLACEMENT_3D('',#30301,#24555,#24556);
#20465=AXIS2_PLACEMENT_3D('',#30303,#24557,#24558);
#20466=AXIS2_PLACEMENT_3D('',#30306,#24560,#24561);
#20467=AXIS2_PLACEMENT_3D('',#30307,#24562,#24563);
#20468=AXIS2_PLACEMENT_3D('',#30309,#24564,#24565);
#20469=AXIS2_PLACEMENT_3D('',#30312,#24567,#24568);
#20470=AXIS2_PLACEMENT_3D('',#30313,#24569,#24570);
#20471=AXIS2_PLACEMENT_3D('',#30315,#24571,#24572);
#20472=AXIS2_PLACEMENT_3D('',#30318,#24574,#24575);
#20473=AXIS2_PLACEMENT_3D('',#30319,#24576,#24577);
#20474=AXIS2_PLACEMENT_3D('',#30321,#24578,#24579);
#20475=AXIS2_PLACEMENT_3D('',#30324,#24581,#24582);
#20476=AXIS2_PLACEMENT_3D('',#30325,#24583,#24584);
#20477=AXIS2_PLACEMENT_3D('',#30327,#24585,#24586);
#20478=AXIS2_PLACEMENT_3D('',#30330,#24588,#24589);
#20479=AXIS2_PLACEMENT_3D('',#30331,#24590,#24591);
#20480=AXIS2_PLACEMENT_3D('',#30333,#24592,#24593);
#20481=AXIS2_PLACEMENT_3D('',#30336,#24595,#24596);
#20482=AXIS2_PLACEMENT_3D('',#30337,#24597,#24598);
#20483=AXIS2_PLACEMENT_3D('',#30346,#24603,#24604);
#20484=AXIS2_PLACEMENT_3D('',#30352,#24608,#24609);
#20485=AXIS2_PLACEMENT_3D('',#30358,#24613,#24614);
#20486=AXIS2_PLACEMENT_3D('',#30361,#24617,#24618);
#20487=AXIS2_PLACEMENT_3D('',#30362,#24619,#24620);
#24469=DIRECTION('axis',(0.,0.,1.));
#24470=DIRECTION('refdir',(1.,0.,0.));
#24471=DIRECTION('center_axis',(0.,0.,1.));
#24472=DIRECTION('ref_axis',(1.,0.,0.));
#24473=DIRECTION('center_axis',(0.,0.,1.));
#24474=DIRECTION('ref_axis',(1.,0.,0.));
#24475=DIRECTION('',(0.,0.,1.));
#24476=DIRECTION('center_axis',(0.,0.,-1.));
#24477=DIRECTION('ref_axis',(1.,0.,0.));
#24478=DIRECTION('center_axis',(0.,0.,1.));
#24479=DIRECTION('ref_axis',(1.,0.,0.));
#24480=DIRECTION('center_axis',(0.,0.,1.));
#24481=DIRECTION('ref_axis',(1.,0.,0.));
#24482=DIRECTION('',(0.,0.,1.));
#24483=DIRECTION('center_axis',(0.,0.,-1.));
#24484=DIRECTION('ref_axis',(1.,0.,0.));
#24485=DIRECTION('center_axis',(0.,0.,1.));
#24486=DIRECTION('ref_axis',(1.,0.,0.));
#24487=DIRECTION('center_axis',(0.,0.,1.));
#24488=DIRECTION('ref_axis',(1.,0.,0.));
#24489=DIRECTION('',(0.,0.,1.));
#24490=DIRECTION('center_axis',(0.,0.,-1.));
#24491=DIRECTION('ref_axis',(1.,0.,0.));
#24492=DIRECTION('center_axis',(0.,0.,1.));
#24493=DIRECTION('ref_axis',(1.,0.,0.));
#24494=DIRECTION('center_axis',(0.,0.,1.));
#24495=DIRECTION('ref_axis',(1.,0.,0.));
#24496=DIRECTION('',(0.,0.,1.));
#24497=DIRECTION('center_axis',(0.,0.,-1.));
#24498=DIRECTION('ref_axis',(1.,0.,0.));
#24499=DIRECTION('center_axis',(0.,0.,1.));
#24500=DIRECTION('ref_axis',(1.,0.,0.));
#24501=DIRECTION('center_axis',(0.,0.,1.));
#24502=DIRECTION('ref_axis',(1.,0.,0.));
#24503=DIRECTION('',(0.,0.,1.));
#24504=DIRECTION('center_axis',(0.,0.,-1.));
#24505=DIRECTION('ref_axis',(1.,0.,0.));
#24506=DIRECTION('center_axis',(0.,0.,1.));
#24507=DIRECTION('ref_axis',(1.,0.,0.));
#24508=DIRECTION('center_axis',(0.,0.,1.));
#24509=DIRECTION('ref_axis',(1.,0.,0.));
#24510=DIRECTION('',(0.,0.,1.));
#24511=DIRECTION('center_axis',(0.,0.,-1.));
#24512=DIRECTION('ref_axis',(1.,0.,0.));
#24513=DIRECTION('center_axis',(0.,0.,1.));
#24514=DIRECTION('ref_axis',(1.,0.,0.));
#24515=DIRECTION('center_axis',(0.,0.,1.));
#24516=DIRECTION('ref_axis',(1.,0.,0.));
#24517=DIRECTION('',(0.,0.,1.));
#24518=DIRECTION('center_axis',(0.,0.,-1.));
#24519=DIRECTION('ref_axis',(1.,0.,0.));
#24520=DIRECTION('center_axis',(0.,0.,1.));
#24521=DIRECTION('ref_axis',(1.,0.,0.));
#24522=DIRECTION('center_axis',(0.,0.,1.));
#24523=DIRECTION('ref_axis',(1.,0.,0.));
#24524=DIRECTION('',(0.,0.,1.));
#24525=DIRECTION('center_axis',(0.,0.,-1.));
#24526=DIRECTION('ref_axis',(1.,0.,0.));
#24527=DIRECTION('center_axis',(0.,0.,1.));
#24528=DIRECTION('ref_axis',(1.,0.,0.));
#24529=DIRECTION('center_axis',(0.,0.,1.));
#24530=DIRECTION('ref_axis',(1.,0.,0.));
#24531=DIRECTION('',(0.,0.,1.));
#24532=DIRECTION('center_axis',(0.,0.,-1.));
#24533=DIRECTION('ref_axis',(1.,0.,0.));
#24534=DIRECTION('center_axis',(0.,0.,1.));
#24535=DIRECTION('ref_axis',(1.,0.,0.));
#24536=DIRECTION('center_axis',(0.,0.,1.));
#24537=DIRECTION('ref_axis',(1.,0.,0.));
#24538=DIRECTION('',(0.,0.,1.));
#24539=DIRECTION('center_axis',(0.,0.,-1.));
#24540=DIRECTION('ref_axis',(1.,0.,0.));
#24541=DIRECTION('center_axis',(0.,0.,1.));
#24542=DIRECTION('ref_axis',(1.,0.,0.));
#24543=DIRECTION('center_axis',(0.,0.,1.));
#24544=DIRECTION('ref_axis',(1.,0.,0.));
#24545=DIRECTION('',(0.,0.,1.));
#24546=DIRECTION('center_axis',(0.,0.,-1.));
#24547=DIRECTION('ref_axis',(1.,0.,0.));
#24548=DIRECTION('center_axis',(0.,0.,1.));
#24549=DIRECTION('ref_axis',(1.,0.,0.));
#24550=DIRECTION('center_axis',(0.,0.,1.));
#24551=DIRECTION('ref_axis',(1.,0.,0.));
#24552=DIRECTION('',(0.,0.,1.));
#24553=DIRECTION('center_axis',(0.,0.,-1.));
#24554=DIRECTION('ref_axis',(1.,0.,0.));
#24555=DIRECTION('center_axis',(0.,0.,1.));
#24556=DIRECTION('ref_axis',(1.,0.,0.));
#24557=DIRECTION('center_axis',(0.,0.,1.));
#24558=DIRECTION('ref_axis',(1.,0.,0.));
#24559=DIRECTION('',(0.,0.,1.));
#24560=DIRECTION('center_axis',(0.,0.,-1.));
#24561=DIRECTION('ref_axis',(1.,0.,0.));
#24562=DIRECTION('center_axis',(0.,0.,1.));
#24563=DIRECTION('ref_axis',(1.,0.,0.));
#24564=DIRECTION('center_axis',(0.,0.,1.));
#24565=DIRECTION('ref_axis',(1.,0.,0.));
#24566=DIRECTION('',(0.,0.,1.));
#24567=DIRECTION('center_axis',(0.,0.,-1.));
#24568=DIRECTION('ref_axis',(1.,0.,0.));
#24569=DIRECTION('center_axis',(0.,0.,1.));
#24570=DIRECTION('ref_axis',(1.,0.,0.));
#24571=DIRECTION('center_axis',(0.,0.,1.));
#24572=DIRECTION('ref_axis',(1.,0.,0.));
#24573=DIRECTION('',(0.,0.,1.));
#24574=DIRECTION('center_axis',(0.,0.,-1.));
#24575=DIRECTION('ref_axis',(1.,0.,0.));
#24576=DIRECTION('center_axis',(0.,0.,1.));
#24577=DIRECTION('ref_axis',(1.,0.,0.));
#24578=DIRECTION('center_axis',(0.,0.,1.));
#24579=DIRECTION('ref_axis',(1.,0.,0.));
#24580=DIRECTION('',(0.,0.,1.));
#24581=DIRECTION('center_axis',(0.,0.,-1.));
#24582=DIRECTION('ref_axis',(1.,0.,0.));
#24583=DIRECTION('center_axis',(0.,0.,1.));
#24584=DIRECTION('ref_axis',(1.,0.,0.));
#24585=DIRECTION('center_axis',(0.,0.,1.));
#24586=DIRECTION('ref_axis',(1.,0.,0.));
#24587=DIRECTION('',(0.,0.,1.));
#24588=DIRECTION('center_axis',(0.,0.,-1.));
#24589=DIRECTION('ref_axis',(1.,0.,0.));
#24590=DIRECTION('center_axis',(0.,0.,1.));
#24591=DIRECTION('ref_axis',(1.,0.,0.));
#24592=DIRECTION('center_axis',(0.,0.,1.));
#24593=DIRECTION('ref_axis',(1.,0.,0.));
#24594=DIRECTION('',(0.,0.,1.));
#24595=DIRECTION('center_axis',(0.,0.,-1.));
#24596=DIRECTION('ref_axis',(1.,0.,0.));
#24597=DIRECTION('center_axis',(0.,1.,0.));
#24598=DIRECTION('ref_axis',(-1.,0.,0.));
#24599=DIRECTION('',(-1.,0.,0.));
#24600=DIRECTION('',(0.,0.,1.));
#24601=DIRECTION('',(-1.,0.,0.));
#24602=DIRECTION('',(0.,0.,1.));
#24603=DIRECTION('center_axis',(1.,0.,0.));
#24604=DIRECTION('ref_axis',(0.,1.,0.));
#24605=DIRECTION('',(0.,1.,0.));
#24606=DIRECTION('',(0.,1.,0.));
#24607=DIRECTION('',(0.,0.,1.));
#24608=DIRECTION('center_axis',(0.,-1.,0.));
#24609=DIRECTION('ref_axis',(1.,0.,0.));
#24610=DIRECTION('',(1.,0.,0.));
#24611=DIRECTION('',(1.,0.,0.));
#24612=DIRECTION('',(0.,0.,1.));
#24613=DIRECTION('center_axis',(-1.,0.,0.));
#24614=DIRECTION('ref_axis',(0.,-1.,0.));
#24615=DIRECTION('',(0.,-1.,0.));
#24616=DIRECTION('',(0.,-1.,0.));
#24617=DIRECTION('center_axis',(0.,0.,1.));
#24618=DIRECTION('ref_axis',(1.,0.,0.));
#24619=DIRECTION('center_axis',(0.,0.,1.));
#24620=DIRECTION('ref_axis',(1.,0.,0.));
#30228=CARTESIAN_POINT('',(0.,0.,0.));
#30229=CARTESIAN_POINT('Origin',(7.2,-0.35,15.));
#30230=CARTESIAN_POINT('',(7.035,-0.35,15.1));
#30231=CARTESIAN_POINT('Origin',(7.2,-0.35,15.1));
#30232=CARTESIAN_POINT('',(7.035,-0.35,16.3));
#30233=CARTESIAN_POINT('',(7.035,-0.35,15.));
#30234=CARTESIAN_POINT('Origin',(7.2,-0.35,16.3));
#30235=CARTESIAN_POINT('Origin',(7.2,0.35,15.));
#30236=CARTESIAN_POINT('',(7.035,0.35,15.1));
#30237=CARTESIAN_POINT('Origin',(7.2,0.35,15.1));
#30238=CARTESIAN_POINT('',(7.035,0.35,16.3));
#30239=CARTESIAN_POINT('',(7.035,0.35,15.));
#30240=CARTESIAN_POINT('Origin',(7.2,0.35,16.3));
#30241=CARTESIAN_POINT('Origin',(-2.,-1.5,15.));
#30242=CARTESIAN_POINT('',(-2.225,-1.5,15.1));
#30243=CARTESIAN_POINT('Origin',(-2.,-1.5,15.1));
#30244=CARTESIAN_POINT('',(-2.225,-1.5,16.3));
#30245=CARTESIAN_POINT('',(-2.225,-1.5,15.));
#30246=CARTESIAN_POINT('Origin',(-2.,-1.5,16.3));
#30247=CARTESIAN_POINT('Origin',(2.,-1.5,15.));
#30248=CARTESIAN_POINT('',(1.775,-1.5,15.1));
#30249=CARTESIAN_POINT('Origin',(2.,-1.5,15.1));
#30250=CARTESIAN_POINT('',(1.775,-1.5,16.3));
#30251=CARTESIAN_POINT('',(1.775,-1.5,15.));
#30252=CARTESIAN_POINT('Origin',(2.,-1.5,16.3));
#30253=CARTESIAN_POINT('Origin',(0.,3.5,15.));
#30254=CARTESIAN_POINT('',(-0.225,3.5,15.1));
#30255=CARTESIAN_POINT('Origin',(0.,3.5,15.1));
#30256=CARTESIAN_POINT('',(-0.225,3.5,16.3));
#30257=CARTESIAN_POINT('',(-0.225,3.5,15.));
#30258=CARTESIAN_POINT('Origin',(0.,3.5,16.3));
#30259=CARTESIAN_POINT('Origin',(0.,6.5,15.));
#30260=CARTESIAN_POINT('',(-0.225,6.5,15.1));
#30261=CARTESIAN_POINT('Origin',(0.,6.5,15.1));
#30262=CARTESIAN_POINT('',(-0.225,6.5,16.3));
#30263=CARTESIAN_POINT('',(-0.225,6.5,15.));
#30264=CARTESIAN_POINT('Origin',(0.,6.5,16.3));
#30265=CARTESIAN_POINT('Origin',(-1.5,5.,15.));
#30266=CARTESIAN_POINT('',(-1.725,5.,15.1));
#30267=CARTESIAN_POINT('Origin',(-1.5,5.,15.1));
#30268=CARTESIAN_POINT('',(-1.725,5.,16.3));
#30269=CARTESIAN_POINT('',(-1.725,5.,15.));
#30270=CARTESIAN_POINT('Origin',(-1.5,5.,16.3));
#30271=CARTESIAN_POINT('Origin',(4.86862915010152,-1.13137084989848,15.));
#30272=CARTESIAN_POINT('',(4.64362915010152,-1.13137084989848,15.1));
#30273=CARTESIAN_POINT('Origin',(4.86862915010152,-1.13137084989848,15.1));
#30274=CARTESIAN_POINT('',(4.64362915010152,-1.13137084989848,16.3));
#30275=CARTESIAN_POINT('',(4.64362915010152,-1.13137084989848,15.));
#30276=CARTESIAN_POINT('Origin',(4.86862915010152,-1.13137084989848,16.3));
#30277=CARTESIAN_POINT('Origin',(4.86862915010152,1.13137084989848,15.));
#30278=CARTESIAN_POINT('',(4.64362915010152,1.13137084989848,15.1));
#30279=CARTESIAN_POINT('Origin',(4.86862915010152,1.13137084989848,15.1));
#30280=CARTESIAN_POINT('',(4.64362915010152,1.13137084989848,16.3));
#30281=CARTESIAN_POINT('',(4.64362915010152,1.13137084989848,15.));
#30282=CARTESIAN_POINT('Origin',(4.86862915010152,1.13137084989848,16.3));
#30283=CARTESIAN_POINT('Origin',(7.13137084989848,1.13137084989848,15.));
#30284=CARTESIAN_POINT('',(6.90637084989848,1.13137084989848,15.1));
#30285=CARTESIAN_POINT('Origin',(7.13137084989848,1.13137084989848,15.1));
#30286=CARTESIAN_POINT('',(6.90637084989848,1.13137084989848,16.3));
#30287=CARTESIAN_POINT('',(6.90637084989848,1.13137084989848,15.));
#30288=CARTESIAN_POINT('Origin',(7.13137084989848,1.13137084989848,16.3));
#30289=CARTESIAN_POINT('Origin',(7.13137084989848,-1.13137084989848,15.));
#30290=CARTESIAN_POINT('',(6.90637084989848,-1.13137084989848,15.1));
#30291=CARTESIAN_POINT('Origin',(7.13137084989848,-1.13137084989848,15.1));
#30292=CARTESIAN_POINT('',(6.90637084989848,-1.13137084989848,16.3));
#30293=CARTESIAN_POINT('',(6.90637084989848,-1.13137084989848,15.));
#30294=CARTESIAN_POINT('Origin',(7.13137084989848,-1.13137084989848,16.3));
#30295=CARTESIAN_POINT('Origin',(-7.13137084989848,-1.13137084989848,15.));
#30296=CARTESIAN_POINT('',(-7.35637084989848,-1.13137084989848,15.1));
#30297=CARTESIAN_POINT('Origin',(-7.13137084989848,-1.13137084989848,15.1));
#30298=CARTESIAN_POINT('',(-7.35637084989848,-1.13137084989848,16.3));
#30299=CARTESIAN_POINT('',(-7.35637084989848,-1.13137084989848,15.));
#30300=CARTESIAN_POINT('Origin',(-7.13137084989848,-1.13137084989848,16.3));
#30301=CARTESIAN_POINT('Origin',(-7.13137084989848,1.13137084989848,15.));
#30302=CARTESIAN_POINT('',(-7.35637084989848,1.13137084989848,15.1));
#30303=CARTESIAN_POINT('Origin',(-7.13137084989848,1.13137084989848,15.1));
#30304=CARTESIAN_POINT('',(-7.35637084989848,1.13137084989848,16.3));
#30305=CARTESIAN_POINT('',(-7.35637084989848,1.13137084989848,15.));
#30306=CARTESIAN_POINT('Origin',(-7.13137084989848,1.13137084989848,16.3));
#30307=CARTESIAN_POINT('Origin',(-4.86862915010152,1.13137084989848,15.));
#30308=CARTESIAN_POINT('',(-5.09362915010152,1.13137084989848,15.1));
#30309=CARTESIAN_POINT('Origin',(-4.86862915010152,1.13137084989848,15.1));
#30310=CARTESIAN_POINT('',(-5.09362915010152,1.13137084989848,16.3));
#30311=CARTESIAN_POINT('',(-5.09362915010152,1.13137084989848,15.));
#30312=CARTESIAN_POINT('Origin',(-4.86862915010152,1.13137084989848,16.3));
#30313=CARTESIAN_POINT('Origin',(-4.86862915010152,-1.13137084989848,15.));
#30314=CARTESIAN_POINT('',(-5.09362915010152,-1.13137084989848,15.1));
#30315=CARTESIAN_POINT('Origin',(-4.86862915010152,-1.13137084989848,15.1));
#30316=CARTESIAN_POINT('',(-5.09362915010152,-1.13137084989848,16.3));
#30317=CARTESIAN_POINT('',(-5.09362915010152,-1.13137084989848,15.));
#30318=CARTESIAN_POINT('Origin',(-4.86862915010152,-1.13137084989848,16.3));
#30319=CARTESIAN_POINT('Origin',(0.,5.,15.));
#30320=CARTESIAN_POINT('',(-0.625,5.,15.1));
#30321=CARTESIAN_POINT('Origin',(0.,5.,15.1));
#30322=CARTESIAN_POINT('',(-0.625,5.,16.3));
#30323=CARTESIAN_POINT('',(-0.625,5.,15.));
#30324=CARTESIAN_POINT('Origin',(0.,5.,16.3));
#30325=CARTESIAN_POINT('Origin',(-6.,0.,15.));
#30326=CARTESIAN_POINT('',(-6.625,-7.65404249467096E-17,15.1));
#30327=CARTESIAN_POINT('Origin',(-6.,0.,15.1));
#30328=CARTESIAN_POINT('',(-6.625,7.65404249467096E-17,16.3));
#30329=CARTESIAN_POINT('',(-6.625,-7.65404249467096E-17,15.));
#30330=CARTESIAN_POINT('Origin',(-6.,0.,16.3));
#30331=CARTESIAN_POINT('Origin',(6.,0.,15.));
#30332=CARTESIAN_POINT('',(5.375,-7.65404249467096E-17,15.1));
#30333=CARTESIAN_POINT('Origin',(6.,0.,15.1));
#30334=CARTESIAN_POINT('',(5.375,7.65404249467096E-17,16.3));
#30335=CARTESIAN_POINT('',(5.375,-7.65404249467096E-17,15.));
#30336=CARTESIAN_POINT('Origin',(6.,0.,16.3));
#30337=CARTESIAN_POINT('Origin',(7.5,7.5,15.1));
#30338=CARTESIAN_POINT('',(7.5,7.5,15.1));
#30339=CARTESIAN_POINT('',(-7.5,7.5,15.1));
#30340=CARTESIAN_POINT('',(7.5,7.5,15.1));
#30341=CARTESIAN_POINT('',(-7.5,7.5,16.3));
#30342=CARTESIAN_POINT('',(-7.5,7.5,15.1));
#30343=CARTESIAN_POINT('',(7.5,7.5,16.3));
#30344=CARTESIAN_POINT('',(7.5,7.5,16.3));
#30345=CARTESIAN_POINT('',(7.5,7.5,15.1));
#30346=CARTESIAN_POINT('Origin',(7.5,-3.5,15.1));
#30347=CARTESIAN_POINT('',(7.5,-3.5,15.1));
#30348=CARTESIAN_POINT('',(7.5,-3.5,15.1));
#30349=CARTESIAN_POINT('',(7.5,-3.5,16.3));
#30350=CARTESIAN_POINT('',(7.5,-3.5,16.3));
#30351=CARTESIAN_POINT('',(7.5,-3.5,15.1));
#30352=CARTESIAN_POINT('Origin',(-7.5,-3.5,15.1));
#30353=CARTESIAN_POINT('',(-7.5,-3.5,15.1));
#30354=CARTESIAN_POINT('',(-7.5,-3.5,15.1));
#30355=CARTESIAN_POINT('',(-7.5,-3.5,16.3));
#30356=CARTESIAN_POINT('',(-7.5,-3.5,16.3));
#30357=CARTESIAN_POINT('',(-7.5,-3.5,15.1));
#30358=CARTESIAN_POINT('Origin',(-7.5,7.5,15.1));
#30359=CARTESIAN_POINT('',(-7.5,7.5,15.1));
#30360=CARTESIAN_POINT('',(-7.5,7.5,16.3));
#30361=CARTESIAN_POINT('Origin',(0.,2.,16.3));
#30362=CARTESIAN_POINT('Origin',(0.,2.,15.1));
#43430=UNCERTAINTY_MEASURE_WITH_UNIT(LENGTH_MEASURE(0.001),#43522,
'DISTANCE_ACCURACY_VALUE',
'Maximum model space distance between geometric entities at asserted c
onnectivities');
#43453=UNCERTAINTY_MEASURE_WITH_UNIT(LENGTH_MEASURE(0.001),#43522,
'DISTANCE_ACCURACY_VALUE',
'Maximum model space distance between geometric entities at asserted c
onnectivities');
#43498=(
GEOMETRIC_REPRESENTATION_CONTEXT(3)
GLOBAL_UNCERTAINTY_ASSIGNED_CONTEXT((#43430))
GLOBAL_UNIT_ASSIGNED_CONTEXT((#43522,#43524,#43525))
REPRESENTATION_CONTEXT('','3D')
);
#43521=(
GEOMETRIC_REPRESENTATION_CONTEXT(3)
GLOBAL_UNCERTAINTY_ASSIGNED_CONTEXT((#43453))
GLOBAL_UNIT_ASSIGNED_CONTEXT((#43522,#43524,#43525))
REPRESENTATION_CONTEXT('','3D')
);
#43522=(
LENGTH_UNIT()
NAMED_UNIT(*)
SI_UNIT(.CENTI.,.METRE.)
);
#43524=(
NAMED_UNIT(*)
PLANE_ANGLE_UNIT()
SI_UNIT($,.RADIAN.)
);
#43525=(
NAMED_UNIT(*)
SI_UNIT($,.STERADIAN.)
SOLID_ANGLE_UNIT()
);
#43570=SHAPE_DEFINITION_REPRESENTATION(#43647,#43838);
#43647=PRODUCT_DEFINITION_SHAPE('',$,#43906);
#43838=SHAPE_REPRESENTATION('',(#20427),#43498);
#43861=PRODUCT_DEFINITION_CONTEXT('part definition',#44064,'design');
#43906=PRODUCT_DEFINITION('Platform','Platform',#43973,#43861);
#43973=PRODUCT_DEFINITION_FORMATION('',$,#44110);
#44064=APPLICATION_CONTEXT(
'Core Data for Automotive Mechanical Design Process');
#44065=PRODUCT_CONTEXT('part definition',#44064,'mechanical');
#44110=PRODUCT('Platform','Platform','Platform',(#44065));
#44182=COLOUR_RGB('Light Blue',0.38,0.62,0.78);
#44183=FILL_AREA_STYLE_COLOUR('',#44182);
#44184=FILL_AREA_STYLE('',(#44183));
#44185=SURFACE_STYLE_FILL_AREA(#44184);
#44186=SURFACE_SIDE_STYLE('',(#44185));
#44187=SURFACE_STYLE_USAGE(.BOTH.,#44186);
#44188=PRESENTATION_STYLE_ASSIGNMENT((#44187));
ENDSEC;
END-ISO-10303-21;
